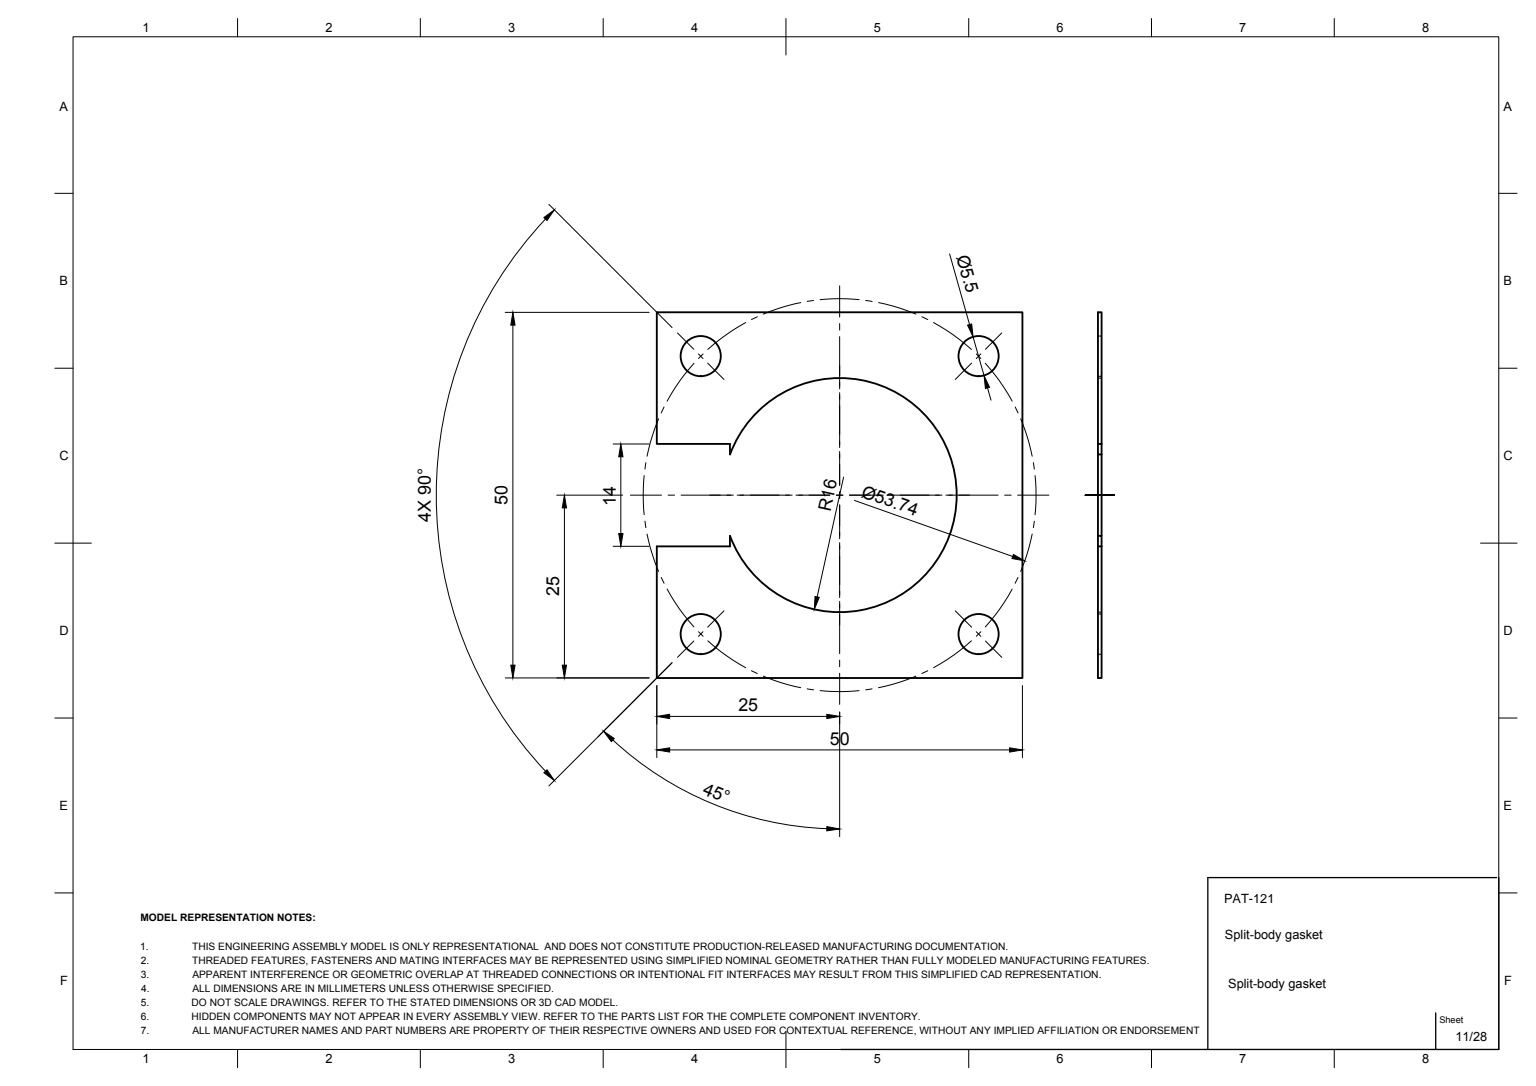
ISO-10303-21;
HEADER;
/* Generated by software containing ST-Developer
 * from STEP Tools, Inc. (www.steptools.com) 
 */

FILE_DESCRIPTION(
/* description */ ('Wall-mounted air drop station'),
/* implementation_level */ '2;1');

FILE_NAME(
/* name */ 'Split-body gasket.step',
/* time_stamp */ '2026-10-28T22:16:19-07:00',
/* author */ (''),
/* organization */ (''),
/* preprocessor_version */ 'ST-DEVELOPER v20.2',
/* originating_system */ 'Autodesk Translation Framework v15.17.0.0',
/* authorisation */ '');

FILE_SCHEMA (('AUTOMOTIVE_DESIGN { 1 0 10303 214 3 1 1 }'));
ENDSEC;

DATA;
#10=MECHANICAL_DESIGN_GEOMETRIC_PRESENTATION_REPRESENTATION('',(#351),#10517);
#293=SHAPE_REPRESENTATION_RELATIONSHIP('SRR','None',#10650,#322);
#322=ADVANCED_BREP_SHAPE_REPRESENTATION('',(#380),#10494);
#351=STYLED_ITEM('',(#10853),#380);
#380=MANIFOLD_SOLID_BREP('Body1',#5890);
#463=FACE_BOUND('',#1308,.T.);
#464=FACE_BOUND('',#1309,.T.);
#465=FACE_BOUND('',#1310,.T.);
#466=FACE_BOUND('',#1311,.T.);
#467=FACE_BOUND('',#1319,.T.);
#468=FACE_BOUND('',#1320,.T.);
#469=FACE_BOUND('',#1321,.T.);
#470=FACE_BOUND('',#1322,.T.);
#602=PLANE('',#6480);
#603=PLANE('',#6481);
#604=PLANE('',#6482);
#605=PLANE('',#6483);
#606=PLANE('',#6484);
#607=PLANE('',#6486);
#608=PLANE('',#6487);
#609=PLANE('',#6490);
#610=PLANE('',#6491);
#611=PLANE('',#6492);
#612=PLANE('',#6493);
#880=FACE_OUTER_BOUND('',#1299,.T.);
#881=FACE_OUTER_BOUND('',#1300,.T.);
#882=FACE_OUTER_BOUND('',#1301,.T.);
#883=FACE_OUTER_BOUND('',#1302,.T.);
#884=FACE_OUTER_BOUND('',#1303,.T.);
#885=FACE_OUTER_BOUND('',#1304,.T.);
#886=FACE_OUTER_BOUND('',#1305,.T.);
#887=FACE_OUTER_BOUND('',#1306,.T.);
#888=FACE_OUTER_BOUND('',#1307,.T.);
#889=FACE_OUTER_BOUND('',#1312,.T.);
#890=FACE_OUTER_BOUND('',#1313,.T.);
#891=FACE_OUTER_BOUND('',#1314,.T.);
#892=FACE_OUTER_BOUND('',#1315,.T.);
#893=FACE_OUTER_BOUND('',#1316,.T.);
#894=FACE_OUTER_BOUND('',#1317,.T.);
#895=FACE_OUTER_BOUND('',#1318,.T.);
#1299=EDGE_LOOP('',(#4507,#4508,#4509,#4510));
#1300=EDGE_LOOP('',(#4511,#4512,#4513,#4514));
#1301=EDGE_LOOP('',(#4515,#4516,#4517,#4518));
#1302=EDGE_LOOP('',(#4519,#4520,#4521,#4522));
#1303=EDGE_LOOP('',(#4523,#4524,#4525,#4526));
#1304=EDGE_LOOP('',(#4527,#4528,#4529,#4530));
#1305=EDGE_LOOP('',(#4531,#4532,#4533,#4534));
#1306=EDGE_LOOP('',(#4535,#4536,#4537,#4538));
#1307=EDGE_LOOP('',(#4539,#4540,#4541,#4542,#4543,#4544,#4545,#4546,#4547,
#4548));
#1308=EDGE_LOOP('',(#4549));
#1309=EDGE_LOOP('',(#4550));
#1310=EDGE_LOOP('',(#4551));
#1311=EDGE_LOOP('',(#4552));
#1312=EDGE_LOOP('',(#4553,#4554,#4555,#4556));
#1313=EDGE_LOOP('',(#4557,#4558,#4559,#4560));
#1314=EDGE_LOOP('',(#4561,#4562,#4563,#4564));
#1315=EDGE_LOOP('',(#4565,#4566,#4567,#4568));
#1316=EDGE_LOOP('',(#4569,#4570,#4571,#4572));
#1317=EDGE_LOOP('',(#4573,#4574,#4575,#4576));
#1318=EDGE_LOOP('',(#4577,#4578,#4579,#4580,#4581,#4582,#4583,#4584,#4585,
#4586));
#1319=EDGE_LOOP('',(#4587));
#1320=EDGE_LOOP('',(#4588));
#1321=EDGE_LOOP('',(#4589));
#1322=EDGE_LOOP('',(#4590));
#1761=LINE('',#9350,#2225);
#1762=LINE('',#9356,#2226);
#1763=LINE('',#9362,#2227);
#1764=LINE('',#9368,#2228);
#1765=LINE('',#9373,#2229);
#1766=LINE('',#9375,#2230);
#1767=LINE('',#9377,#2231);
#1768=LINE('',#9378,#2232);
#1769=LINE('',#9382,#2233);
#1770=LINE('',#9384,#2234);
#1771=LINE('',#9386,#2235);
#1772=LINE('',#9387,#2236);
#1773=LINE('',#9390,#2237);
#1774=LINE('',#9392,#2238);
#1775=LINE('',#9393,#2239);
#1776=LINE('',#9396,#2240);
#1777=LINE('',#9398,#2241);
#1778=LINE('',#9399,#2242);
#1779=LINE('',#9403,#2243);
#1780=LINE('',#9405,#2244);
#1781=LINE('',#9407,#2245);
#1782=LINE('',#9409,#2246);
#1783=LINE('',#9410,#2247);
#1784=LINE('',#9413,#2248);
#1785=LINE('',#9414,#2249);
#1786=LINE('',#9417,#2250);
#1787=LINE('',#9418,#2251);
#1788=LINE('',#9423,#2252);
#1789=LINE('',#9424,#2253);
#1790=LINE('',#9427,#2254);
#1791=LINE('',#9428,#2255);
#1792=LINE('',#9430,#2256);
#2225=VECTOR('',#7563,0.275);
#2226=VECTOR('',#7570,0.275);
#2227=VECTOR('',#7577,0.275);
#2228=VECTOR('',#7584,0.275);
#2229=VECTOR('',#7589,1.);
#2230=VECTOR('',#7590,1.);
#2231=VECTOR('',#7591,1.);
#2232=VECTOR('',#7592,1.);
#2233=VECTOR('',#7595,1.);
#2234=VECTOR('',#7596,1.);
#2235=VECTOR('',#7597,1.);
#2236=VECTOR('',#7598,1.);
#2237=VECTOR('',#7601,1.);
#2238=VECTOR('',#7602,1.);
#2239=VECTOR('',#7603,1.);
#2240=VECTOR('',#7606,1.);
#2241=VECTOR('',#7607,1.);
#2242=VECTOR('',#7608,1.);
#2243=VECTOR('',#7613,1.);
#2244=VECTOR('',#7614,1.);
#2245=VECTOR('',#7615,1.);
#2246=VECTOR('',#7616,1.);
#2247=VECTOR('',#7617,1.);
#2248=VECTOR('',#7620,1.);
#2249=VECTOR('',#7621,1.);
#2250=VECTOR('',#7624,1.);
#2251=VECTOR('',#7625,1.);
#2252=VECTOR('',#7632,1.);
#2253=VECTOR('',#7633,1.);
#2254=VECTOR('',#7636,1.);
#2255=VECTOR('',#7637,1.);
#2256=VECTOR('',#7640,1.);
#2618=CIRCLE('',#6469,0.275);
#2619=CIRCLE('',#6470,0.275);
#2620=CIRCLE('',#6472,0.275);
#2621=CIRCLE('',#6473,0.275);
#2622=CIRCLE('',#6475,0.275);
#2623=CIRCLE('',#6476,0.275);
#2624=CIRCLE('',#6478,0.275);
#2625=CIRCLE('',#6479,0.275);
#2626=CIRCLE('',#6485,1.6);
#2627=CIRCLE('',#6489,1.6);
#2943=VERTEX_POINT('',#9347);
#2944=VERTEX_POINT('',#9349);
#2945=VERTEX_POINT('',#9353);
#2946=VERTEX_POINT('',#9355);
#2947=VERTEX_POINT('',#9359);
#2948=VERTEX_POINT('',#9361);
#2949=VERTEX_POINT('',#9365);
#2950=VERTEX_POINT('',#9367);
#2951=VERTEX_POINT('',#9371);
#2952=VERTEX_POINT('',#9372);
#2953=VERTEX_POINT('',#9374);
#2954=VERTEX_POINT('',#9376);
#2955=VERTEX_POINT('',#9380);
#2956=VERTEX_POINT('',#9381);
#2957=VERTEX_POINT('',#9383);
#2958=VERTEX_POINT('',#9385);
#2959=VERTEX_POINT('',#9389);
#2960=VERTEX_POINT('',#9391);
#2961=VERTEX_POINT('',#9395);
#2962=VERTEX_POINT('',#9397);
#2963=VERTEX_POINT('',#9402);
#2964=VERTEX_POINT('',#9404);
#2965=VERTEX_POINT('',#9406);
#2966=VERTEX_POINT('',#9408);
#2967=VERTEX_POINT('',#9412);
#2968=VERTEX_POINT('',#9416);
#2969=VERTEX_POINT('',#9422);
#2970=VERTEX_POINT('',#9426);
#3511=EDGE_CURVE('',#2943,#2943,#2618,.T.);
#3512=EDGE_CURVE('',#2943,#2944,#1761,.T.);
#3513=EDGE_CURVE('',#2944,#2944,#2619,.T.);
#3514=EDGE_CURVE('',#2945,#2945,#2620,.T.);
#3515=EDGE_CURVE('',#2945,#2946,#1762,.T.);
#3516=EDGE_CURVE('',#2946,#2946,#2621,.T.);
#3517=EDGE_CURVE('',#2947,#2947,#2622,.T.);
#3518=EDGE_CURVE('',#2947,#2948,#1763,.T.);
#3519=EDGE_CURVE('',#2948,#2948,#2623,.T.);
#3520=EDGE_CURVE('',#2949,#2949,#2624,.T.);
#3521=EDGE_CURVE('',#2949,#2950,#1764,.T.);
#3522=EDGE_CURVE('',#2950,#2950,#2625,.T.);
#3523=EDGE_CURVE('',#2951,#2952,#1765,.T.);
#3524=EDGE_CURVE('',#2951,#2953,#1766,.T.);
#3525=EDGE_CURVE('',#2954,#2953,#1767,.T.);
#3526=EDGE_CURVE('',#2952,#2954,#1768,.T.);
#3527=EDGE_CURVE('',#2955,#2956,#1769,.T.);
#3528=EDGE_CURVE('',#2955,#2957,#1770,.T.);
#3529=EDGE_CURVE('',#2958,#2957,#1771,.T.);
#3530=EDGE_CURVE('',#2956,#2958,#1772,.T.);
#3531=EDGE_CURVE('',#2959,#2951,#1773,.T.);
#3532=EDGE_CURVE('',#2960,#2959,#1774,.T.);
#3533=EDGE_CURVE('',#2953,#2960,#1775,.T.);
#3534=EDGE_CURVE('',#2961,#2955,#1776,.T.);
#3535=EDGE_CURVE('',#2962,#2961,#1777,.T.);
#3536=EDGE_CURVE('',#2957,#2962,#1778,.T.);
#3537=EDGE_CURVE('',#2960,#2958,#2626,.T.);
#3538=EDGE_CURVE('',#2962,#2963,#1779,.T.);
#3539=EDGE_CURVE('',#2963,#2964,#1780,.T.);
#3540=EDGE_CURVE('',#2964,#2965,#1781,.T.);
#3541=EDGE_CURVE('',#2965,#2966,#1782,.T.);
#3542=EDGE_CURVE('',#2966,#2954,#1783,.T.);
#3543=EDGE_CURVE('',#2967,#2961,#1784,.T.);
#3544=EDGE_CURVE('',#2967,#2963,#1785,.T.);
#3545=EDGE_CURVE('',#2968,#2966,#1786,.T.);
#3546=EDGE_CURVE('',#2952,#2968,#1787,.T.);
#3547=EDGE_CURVE('',#2956,#2959,#2627,.T.);
#3548=EDGE_CURVE('',#2968,#2969,#1788,.T.);
#3549=EDGE_CURVE('',#2969,#2965,#1789,.T.);
#3550=EDGE_CURVE('',#2969,#2970,#1790,.T.);
#3551=EDGE_CURVE('',#2970,#2964,#1791,.T.);
#3552=EDGE_CURVE('',#2970,#2967,#1792,.T.);
#4507=ORIENTED_EDGE('',*,*,#3511,.F.);
#4508=ORIENTED_EDGE('',*,*,#3512,.T.);
#4509=ORIENTED_EDGE('',*,*,#3513,.F.);
#4510=ORIENTED_EDGE('',*,*,#3512,.F.);
#4511=ORIENTED_EDGE('',*,*,#3514,.F.);
#4512=ORIENTED_EDGE('',*,*,#3515,.T.);
#4513=ORIENTED_EDGE('',*,*,#3516,.F.);
#4514=ORIENTED_EDGE('',*,*,#3515,.F.);
#4515=ORIENTED_EDGE('',*,*,#3517,.F.);
#4516=ORIENTED_EDGE('',*,*,#3518,.T.);
#4517=ORIENTED_EDGE('',*,*,#3519,.F.);
#4518=ORIENTED_EDGE('',*,*,#3518,.F.);
#4519=ORIENTED_EDGE('',*,*,#3520,.F.);
#4520=ORIENTED_EDGE('',*,*,#3521,.T.);
#4521=ORIENTED_EDGE('',*,*,#3522,.F.);
#4522=ORIENTED_EDGE('',*,*,#3521,.F.);
#4523=ORIENTED_EDGE('',*,*,#3523,.F.);
#4524=ORIENTED_EDGE('',*,*,#3524,.T.);
#4525=ORIENTED_EDGE('',*,*,#3525,.F.);
#4526=ORIENTED_EDGE('',*,*,#3526,.F.);
#4527=ORIENTED_EDGE('',*,*,#3527,.F.);
#4528=ORIENTED_EDGE('',*,*,#3528,.T.);
#4529=ORIENTED_EDGE('',*,*,#3529,.F.);
#4530=ORIENTED_EDGE('',*,*,#3530,.F.);
#4531=ORIENTED_EDGE('',*,*,#3531,.F.);
#4532=ORIENTED_EDGE('',*,*,#3532,.F.);
#4533=ORIENTED_EDGE('',*,*,#3533,.F.);
#4534=ORIENTED_EDGE('',*,*,#3524,.F.);
#4535=ORIENTED_EDGE('',*,*,#3534,.F.);
#4536=ORIENTED_EDGE('',*,*,#3535,.F.);
#4537=ORIENTED_EDGE('',*,*,#3536,.F.);
#4538=ORIENTED_EDGE('',*,*,#3528,.F.);
#4539=ORIENTED_EDGE('',*,*,#3525,.T.);
#4540=ORIENTED_EDGE('',*,*,#3533,.T.);
#4541=ORIENTED_EDGE('',*,*,#3537,.T.);
#4542=ORIENTED_EDGE('',*,*,#3529,.T.);
#4543=ORIENTED_EDGE('',*,*,#3536,.T.);
#4544=ORIENTED_EDGE('',*,*,#3538,.T.);
#4545=ORIENTED_EDGE('',*,*,#3539,.T.);
#4546=ORIENTED_EDGE('',*,*,#3540,.T.);
#4547=ORIENTED_EDGE('',*,*,#3541,.T.);
#4548=ORIENTED_EDGE('',*,*,#3542,.T.);
#4549=ORIENTED_EDGE('',*,*,#3513,.T.);
#4550=ORIENTED_EDGE('',*,*,#3516,.T.);
#4551=ORIENTED_EDGE('',*,*,#3519,.T.);
#4552=ORIENTED_EDGE('',*,*,#3522,.T.);
#4553=ORIENTED_EDGE('',*,*,#3535,.T.);
#4554=ORIENTED_EDGE('',*,*,#3543,.F.);
#4555=ORIENTED_EDGE('',*,*,#3544,.T.);
#4556=ORIENTED_EDGE('',*,*,#3538,.F.);
#4557=ORIENTED_EDGE('',*,*,#3526,.T.);
#4558=ORIENTED_EDGE('',*,*,#3542,.F.);
#4559=ORIENTED_EDGE('',*,*,#3545,.F.);
#4560=ORIENTED_EDGE('',*,*,#3546,.F.);
#4561=ORIENTED_EDGE('',*,*,#3532,.T.);
#4562=ORIENTED_EDGE('',*,*,#3547,.F.);
#4563=ORIENTED_EDGE('',*,*,#3530,.T.);
#4564=ORIENTED_EDGE('',*,*,#3537,.F.);
#4565=ORIENTED_EDGE('',*,*,#3548,.F.);
#4566=ORIENTED_EDGE('',*,*,#3545,.T.);
#4567=ORIENTED_EDGE('',*,*,#3541,.F.);
#4568=ORIENTED_EDGE('',*,*,#3549,.F.);
#4569=ORIENTED_EDGE('',*,*,#3550,.F.);
#4570=ORIENTED_EDGE('',*,*,#3549,.T.);
#4571=ORIENTED_EDGE('',*,*,#3540,.F.);
#4572=ORIENTED_EDGE('',*,*,#3551,.F.);
#4573=ORIENTED_EDGE('',*,*,#3552,.F.);
#4574=ORIENTED_EDGE('',*,*,#3551,.T.);
#4575=ORIENTED_EDGE('',*,*,#3539,.F.);
#4576=ORIENTED_EDGE('',*,*,#3544,.F.);
#4577=ORIENTED_EDGE('',*,*,#3523,.T.);
#4578=ORIENTED_EDGE('',*,*,#3546,.T.);
#4579=ORIENTED_EDGE('',*,*,#3548,.T.);
#4580=ORIENTED_EDGE('',*,*,#3550,.T.);
#4581=ORIENTED_EDGE('',*,*,#3552,.T.);
#4582=ORIENTED_EDGE('',*,*,#3543,.T.);
#4583=ORIENTED_EDGE('',*,*,#3534,.T.);
#4584=ORIENTED_EDGE('',*,*,#3527,.T.);
#4585=ORIENTED_EDGE('',*,*,#3547,.T.);
#4586=ORIENTED_EDGE('',*,*,#3531,.T.);
#4587=ORIENTED_EDGE('',*,*,#3511,.T.);
#4588=ORIENTED_EDGE('',*,*,#3514,.T.);
#4589=ORIENTED_EDGE('',*,*,#3517,.T.);
#4590=ORIENTED_EDGE('',*,*,#3520,.T.);
#5475=CYLINDRICAL_SURFACE('',#6468,0.275);
#5476=CYLINDRICAL_SURFACE('',#6471,0.275);
#5477=CYLINDRICAL_SURFACE('',#6474,0.275);
#5478=CYLINDRICAL_SURFACE('',#6477,0.275);
#5479=CYLINDRICAL_SURFACE('',#6488,1.6);
#5653=ADVANCED_FACE('',(#880),#5475,.F.);
#5654=ADVANCED_FACE('',(#881),#5476,.F.);
#5655=ADVANCED_FACE('',(#882),#5477,.F.);
#5656=ADVANCED_FACE('',(#883),#5478,.F.);
#5657=ADVANCED_FACE('',(#884),#602,.F.);
#5658=ADVANCED_FACE('',(#885),#603,.F.);
#5659=ADVANCED_FACE('',(#886),#604,.F.);
#5660=ADVANCED_FACE('',(#887),#605,.F.);
#5661=ADVANCED_FACE('',(#888,#463,#464,#465,#466),#606,.T.);
#5662=ADVANCED_FACE('',(#889),#607,.T.);
#5663=ADVANCED_FACE('',(#890),#608,.T.);
#5664=ADVANCED_FACE('',(#891),#5479,.F.);
#5665=ADVANCED_FACE('',(#892),#609,.T.);
#5666=ADVANCED_FACE('',(#893),#610,.T.);
#5667=ADVANCED_FACE('',(#894),#611,.T.);
#5668=ADVANCED_FACE('',(#895,#467,#468,#469,#470),#612,.F.);
#5890=CLOSED_SHELL('',(#5653,#5654,#5655,#5656,#5657,#5658,#5659,#5660,
#5661,#5662,#5663,#5664,#5665,#5666,#5667,#5668));
#6467=AXIS2_PLACEMENT_3D('',#9345,#7557,#7558);
#6468=AXIS2_PLACEMENT_3D('',#9346,#7559,#7560);
#6469=AXIS2_PLACEMENT_3D('',#9348,#7561,#7562);
#6470=AXIS2_PLACEMENT_3D('',#9351,#7564,#7565);
#6471=AXIS2_PLACEMENT_3D('',#9352,#7566,#7567);
#6472=AXIS2_PLACEMENT_3D('',#9354,#7568,#7569);
#6473=AXIS2_PLACEMENT_3D('',#9357,#7571,#7572);
#6474=AXIS2_PLACEMENT_3D('',#9358,#7573,#7574);
#6475=AXIS2_PLACEMENT_3D('',#9360,#7575,#7576);
#6476=AXIS2_PLACEMENT_3D('',#9363,#7578,#7579);
#6477=AXIS2_PLACEMENT_3D('',#9364,#7580,#7581);
#6478=AXIS2_PLACEMENT_3D('',#9366,#7582,#7583);
#6479=AXIS2_PLACEMENT_3D('',#9369,#7585,#7586);
#6480=AXIS2_PLACEMENT_3D('',#9370,#7587,#7588);
#6481=AXIS2_PLACEMENT_3D('',#9379,#7593,#7594);
#6482=AXIS2_PLACEMENT_3D('',#9388,#7599,#7600);
#6483=AXIS2_PLACEMENT_3D('',#9394,#7604,#7605);
#6484=AXIS2_PLACEMENT_3D('',#9400,#7609,#7610);
#6485=AXIS2_PLACEMENT_3D('',#9401,#7611,#7612);
#6486=AXIS2_PLACEMENT_3D('',#9411,#7618,#7619);
#6487=AXIS2_PLACEMENT_3D('',#9415,#7622,#7623);
#6488=AXIS2_PLACEMENT_3D('',#9419,#7626,#7627);
#6489=AXIS2_PLACEMENT_3D('',#9420,#7628,#7629);
#6490=AXIS2_PLACEMENT_3D('',#9421,#7630,#7631);
#6491=AXIS2_PLACEMENT_3D('',#9425,#7634,#7635);
#6492=AXIS2_PLACEMENT_3D('',#9429,#7638,#7639);
#6493=AXIS2_PLACEMENT_3D('',#9431,#7641,#7642);
#7557=DIRECTION('axis',(0.,0.,1.));
#7558=DIRECTION('refdir',(1.,0.,0.));
#7559=DIRECTION('center_axis',(0.,1.,0.));
#7560=DIRECTION('ref_axis',(1.,0.,0.));
#7561=DIRECTION('center_axis',(0.,1.,0.));
#7562=DIRECTION('ref_axis',(1.,0.,0.));
#7563=DIRECTION('',(0.,1.,0.));
#7564=DIRECTION('center_axis',(0.,-1.,0.));
#7565=DIRECTION('ref_axis',(1.,0.,0.));
#7566=DIRECTION('center_axis',(0.,1.,0.));
#7567=DIRECTION('ref_axis',(1.,0.,0.));
#7568=DIRECTION('center_axis',(0.,1.,0.));
#7569=DIRECTION('ref_axis',(1.,0.,0.));
#7570=DIRECTION('',(0.,1.,0.));
#7571=DIRECTION('center_axis',(0.,-1.,0.));
#7572=DIRECTION('ref_axis',(1.,0.,0.));
#7573=DIRECTION('center_axis',(0.,1.,0.));
#7574=DIRECTION('ref_axis',(1.,0.,0.));
#7575=DIRECTION('center_axis',(0.,1.,0.));
#7576=DIRECTION('ref_axis',(1.,0.,0.));
#7577=DIRECTION('',(0.,1.,0.));
#7578=DIRECTION('center_axis',(0.,-1.,0.));
#7579=DIRECTION('ref_axis',(1.,0.,0.));
#7580=DIRECTION('center_axis',(0.,1.,0.));
#7581=DIRECTION('ref_axis',(1.,0.,0.));
#7582=DIRECTION('center_axis',(0.,1.,0.));
#7583=DIRECTION('ref_axis',(1.,0.,0.));
#7584=DIRECTION('',(0.,1.,0.));
#7585=DIRECTION('center_axis',(0.,-1.,0.));
#7586=DIRECTION('ref_axis',(1.,0.,0.));
#7587=DIRECTION('center_axis',(-1.,0.,0.));
#7588=DIRECTION('ref_axis',(0.,0.,1.));
#7589=DIRECTION('',(0.,0.,1.));
#7590=DIRECTION('',(0.,1.,0.));
#7591=DIRECTION('',(0.,0.,-1.));
#7592=DIRECTION('',(0.,1.,0.));
#7593=DIRECTION('center_axis',(0.,0.,-1.));
#7594=DIRECTION('ref_axis',(-1.,0.,0.));
#7595=DIRECTION('',(-1.,0.,0.));
#7596=DIRECTION('',(0.,1.,0.));
#7597=DIRECTION('',(1.,0.,0.));
#7598=DIRECTION('',(0.,1.,0.));
#7599=DIRECTION('center_axis',(0.,0.,-1.));
#7600=DIRECTION('ref_axis',(-1.,0.,0.));
#7601=DIRECTION('',(-1.,0.,0.));
#7602=DIRECTION('',(0.,-1.,0.));
#7603=DIRECTION('',(1.,0.,0.));
#7604=DIRECTION('center_axis',(1.,0.,0.));
#7605=DIRECTION('ref_axis',(0.,0.,-1.));
#7606=DIRECTION('',(0.,0.,-1.));
#7607=DIRECTION('',(0.,-1.,0.));
#7608=DIRECTION('',(0.,0.,1.));
#7609=DIRECTION('center_axis',(0.,1.,0.));
#7610=DIRECTION('ref_axis',(0.,0.,1.));
#7611=DIRECTION('center_axis',(0.,-1.,0.));
#7612=DIRECTION('ref_axis',(1.,0.,0.));
#7613=DIRECTION('',(1.,0.,0.));
#7614=DIRECTION('',(0.,0.,-1.));
#7615=DIRECTION('',(-1.,0.,0.));
#7616=DIRECTION('',(0.,0.,1.));
#7617=DIRECTION('',(1.,0.,0.));
#7618=DIRECTION('center_axis',(0.,0.,1.));
#7619=DIRECTION('ref_axis',(1.,0.,0.));
#7620=DIRECTION('',(-1.,0.,0.));
#7621=DIRECTION('',(0.,1.,0.));
#7622=DIRECTION('center_axis',(0.,0.,1.));
#7623=DIRECTION('ref_axis',(1.,0.,0.));
#7624=DIRECTION('',(0.,1.,0.));
#7625=DIRECTION('',(-1.,0.,0.));
#7626=DIRECTION('center_axis',(0.,1.,0.));
#7627=DIRECTION('ref_axis',(-1.83697019872103E-16,0.,-1.));
#7628=DIRECTION('center_axis',(0.,1.,0.));
#7629=DIRECTION('ref_axis',(1.,0.,0.));
#7630=DIRECTION('center_axis',(-1.,0.,0.));
#7631=DIRECTION('ref_axis',(0.,0.,1.));
#7632=DIRECTION('',(0.,0.,-1.));
#7633=DIRECTION('',(0.,1.,0.));
#7634=DIRECTION('center_axis',(0.,0.,-1.));
#7635=DIRECTION('ref_axis',(-1.,0.,0.));
#7636=DIRECTION('',(1.,0.,0.));
#7637=DIRECTION('',(0.,1.,0.));
#7638=DIRECTION('center_axis',(1.,0.,0.));
#7639=DIRECTION('ref_axis',(0.,0.,-1.));
#7640=DIRECTION('',(0.,0.,1.));
#7641=DIRECTION('center_axis',(0.,1.,0.));
#7642=DIRECTION('ref_axis',(1.,0.,0.));
#9345=CARTESIAN_POINT('',(0.,0.,0.));
#9346=CARTESIAN_POINT('Origin',(1.9,-0.1,3.1));
#9347=CARTESIAN_POINT('',(1.625,-0.025,3.1));
#9348=CARTESIAN_POINT('Origin',(1.9,-0.025,3.1));
#9349=CARTESIAN_POINT('',(1.625,0.025,3.1));
#9350=CARTESIAN_POINT('',(1.625,-0.1,3.1));
#9351=CARTESIAN_POINT('Origin',(1.9,0.025,3.1));
#9352=CARTESIAN_POINT('Origin',(-1.9,-0.1,6.9));
#9353=CARTESIAN_POINT('',(-2.175,-0.025,6.9));
#9354=CARTESIAN_POINT('Origin',(-1.9,-0.025,6.9));
#9355=CARTESIAN_POINT('',(-2.175,0.025,6.9));
#9356=CARTESIAN_POINT('',(-2.175,-0.1,6.9));
#9357=CARTESIAN_POINT('Origin',(-1.9,0.025,6.9));
#9358=CARTESIAN_POINT('Origin',(-1.9,-0.1,3.1));
#9359=CARTESIAN_POINT('',(-2.175,-0.025,3.1));
#9360=CARTESIAN_POINT('Origin',(-1.9,-0.025,3.1));
#9361=CARTESIAN_POINT('',(-2.175,0.025,3.1));
#9362=CARTESIAN_POINT('',(-2.175,-0.1,3.1));
#9363=CARTESIAN_POINT('Origin',(-1.9,0.025,3.1));
#9364=CARTESIAN_POINT('Origin',(1.9,-0.1,6.9));
#9365=CARTESIAN_POINT('',(1.625,-0.025,6.9));
#9366=CARTESIAN_POINT('Origin',(1.9,-0.025,6.9));
#9367=CARTESIAN_POINT('',(1.625,0.025,6.9));
#9368=CARTESIAN_POINT('',(1.625,-0.1,6.9));
#9369=CARTESIAN_POINT('Origin',(1.9,0.025,6.9));
#9370=CARTESIAN_POINT('Origin',(-0.7,-0.1,6.5));
#9371=CARTESIAN_POINT('',(-0.7,-0.025,6.5));
#9372=CARTESIAN_POINT('',(-0.7,-0.025,7.5));
#9373=CARTESIAN_POINT('',(-0.7,-0.025,5.75));
#9374=CARTESIAN_POINT('',(-0.7,0.025,6.5));
#9375=CARTESIAN_POINT('',(-0.7,-0.1,6.5));
#9376=CARTESIAN_POINT('',(-0.7,0.025,7.5));
#9377=CARTESIAN_POINT('',(-0.7,0.025,5.75));
#9378=CARTESIAN_POINT('',(-0.7,-0.0625,7.5));
#9379=CARTESIAN_POINT('Origin',(0.7,-0.1,6.5));
#9380=CARTESIAN_POINT('',(0.7,-0.025,6.5));
#9381=CARTESIAN_POINT('',(0.556776436283003,-0.025,6.5));
#9382=CARTESIAN_POINT('',(0.35,-0.025,6.5));
#9383=CARTESIAN_POINT('',(0.7,0.025,6.5));
#9384=CARTESIAN_POINT('',(0.7,-0.1,6.5));
#9385=CARTESIAN_POINT('',(0.556776436283003,0.025,6.5));
#9386=CARTESIAN_POINT('',(0.35,0.025,6.5));
#9387=CARTESIAN_POINT('',(0.556776436283003,-0.1,6.5));
#9388=CARTESIAN_POINT('Origin',(0.7,-0.1,6.5));
#9389=CARTESIAN_POINT('',(-0.556776436283003,-0.025,6.5));
#9390=CARTESIAN_POINT('',(0.35,-0.025,6.5));
#9391=CARTESIAN_POINT('',(-0.556776436283003,0.025,6.5));
#9392=CARTESIAN_POINT('',(-0.556776436283003,-0.1,6.5));
#9393=CARTESIAN_POINT('',(0.35,0.025,6.5));
#9394=CARTESIAN_POINT('Origin',(0.7,-0.1,7.6));
#9395=CARTESIAN_POINT('',(0.7,-0.025,7.5));
#9396=CARTESIAN_POINT('',(0.7,-0.025,6.3));
#9397=CARTESIAN_POINT('',(0.7,0.025,7.5));
#9398=CARTESIAN_POINT('',(0.7,-0.0625,7.5));
#9399=CARTESIAN_POINT('',(0.7,0.025,6.3));
#9400=CARTESIAN_POINT('Origin',(0.,0.025,5.));
#9401=CARTESIAN_POINT('Origin',(0.,0.025,5.));
#9402=CARTESIAN_POINT('',(2.5,0.025,7.5));
#9403=CARTESIAN_POINT('',(2.5,0.025,7.5));
#9404=CARTESIAN_POINT('',(2.5,0.025,2.5));
#9405=CARTESIAN_POINT('',(2.5,0.025,2.5));
#9406=CARTESIAN_POINT('',(-2.5,0.025,2.5));
#9407=CARTESIAN_POINT('',(-2.5,0.025,2.5));
#9408=CARTESIAN_POINT('',(-2.5,0.025,7.5));
#9409=CARTESIAN_POINT('',(-2.5,0.025,7.5));
#9410=CARTESIAN_POINT('',(2.5,0.025,7.5));
#9411=CARTESIAN_POINT('Origin',(-2.5,-0.025,7.5));
#9412=CARTESIAN_POINT('',(2.5,-0.025,7.5));
#9413=CARTESIAN_POINT('',(2.5,-0.025,7.5));
#9414=CARTESIAN_POINT('',(2.5,-0.025,7.5));
#9415=CARTESIAN_POINT('Origin',(-2.5,-0.025,7.5));
#9416=CARTESIAN_POINT('',(-2.5,-0.025,7.5));
#9417=CARTESIAN_POINT('',(-2.5,-0.025,7.5));
#9418=CARTESIAN_POINT('',(2.5,-0.025,7.5));
#9419=CARTESIAN_POINT('Origin',(0.,-0.1,5.));
#9420=CARTESIAN_POINT('Origin',(0.,-0.025,5.));
#9421=CARTESIAN_POINT('Origin',(-2.5,-0.025,2.5));
#9422=CARTESIAN_POINT('',(-2.5,-0.025,2.5));
#9423=CARTESIAN_POINT('',(-2.5,-0.025,7.5));
#9424=CARTESIAN_POINT('',(-2.5,-0.025,2.5));
#9425=CARTESIAN_POINT('Origin',(2.5,-0.025,2.5));
#9426=CARTESIAN_POINT('',(2.5,-0.025,2.5));
#9427=CARTESIAN_POINT('',(-2.5,-0.025,2.5));
#9428=CARTESIAN_POINT('',(2.5,-0.025,2.5));
#9429=CARTESIAN_POINT('Origin',(2.5,-0.025,7.5));
#9430=CARTESIAN_POINT('',(2.5,-0.025,2.5));
#9431=CARTESIAN_POINT('Origin',(0.,-0.025,5.));
#10461=UNCERTAINTY_MEASURE_WITH_UNIT(LENGTH_MEASURE(0.001),#10518,
'DISTANCE_ACCURACY_VALUE',
'Maximum model space distance between geometric entities at asserted c
onnectivities');
#10484=UNCERTAINTY_MEASURE_WITH_UNIT(LENGTH_MEASURE(0.001),#10518,
'DISTANCE_ACCURACY_VALUE',
'Maximum model space distance between geometric entities at asserted c
onnectivities');
#10494=(
GEOMETRIC_REPRESENTATION_CONTEXT(3)
GLOBAL_UNCERTAINTY_ASSIGNED_CONTEXT((#10461))
GLOBAL_UNIT_ASSIGNED_CONTEXT((#10518,#10520,#10521))
REPRESENTATION_CONTEXT('','3D')
);
#10517=(
GEOMETRIC_REPRESENTATION_CONTEXT(3)
GLOBAL_UNCERTAINTY_ASSIGNED_CONTEXT((#10484))
GLOBAL_UNIT_ASSIGNED_CONTEXT((#10518,#10520,#10521))
REPRESENTATION_CONTEXT('','3D')
);
#10518=(
LENGTH_UNIT()
NAMED_UNIT(*)
SI_UNIT(.CENTI.,.METRE.)
);
#10520=(
NAMED_UNIT(*)
PLANE_ANGLE_UNIT()
SI_UNIT($,.RADIAN.)
);
#10521=(
NAMED_UNIT(*)
SI_UNIT($,.STERADIAN.)
SOLID_ANGLE_UNIT()
);
#10531=SHAPE_DEFINITION_REPRESENTATION(#10563,#10650);
#10563=PRODUCT_DEFINITION_SHAPE('',$,#10683);
#10650=SHAPE_REPRESENTATION('',(#6467),#10494);
#10673=PRODUCT_DEFINITION_CONTEXT('part definition',#10771,'design');
#10683=PRODUCT_DEFINITION('Split-body gasket','Split-body gasket',#10715,
#10673);
#10715=PRODUCT_DEFINITION_FORMATION('',$,#10782);
#10771=APPLICATION_CONTEXT(
'Core Data for Automotive Mechanical Design Process');
#10772=PRODUCT_CONTEXT('part definition',#10771,'mechanical');
#10782=PRODUCT('Split-body gasket','Split-body gasket',
'Split-body gasket',(#10772));
#10847=COLOUR_RGB('Dark Blue',0.08,0.2,0.34);
#10848=FILL_AREA_STYLE_COLOUR('',#10847);
#10849=FILL_AREA_STYLE('',(#10848));
#10850=SURFACE_STYLE_FILL_AREA(#10849);
#10851=SURFACE_SIDE_STYLE('',(#10850));
#10852=SURFACE_STYLE_USAGE(.BOTH.,#10851);
#10853=PRESENTATION_STYLE_ASSIGNMENT((#10852));
ENDSEC;
END-ISO-10303-21;
